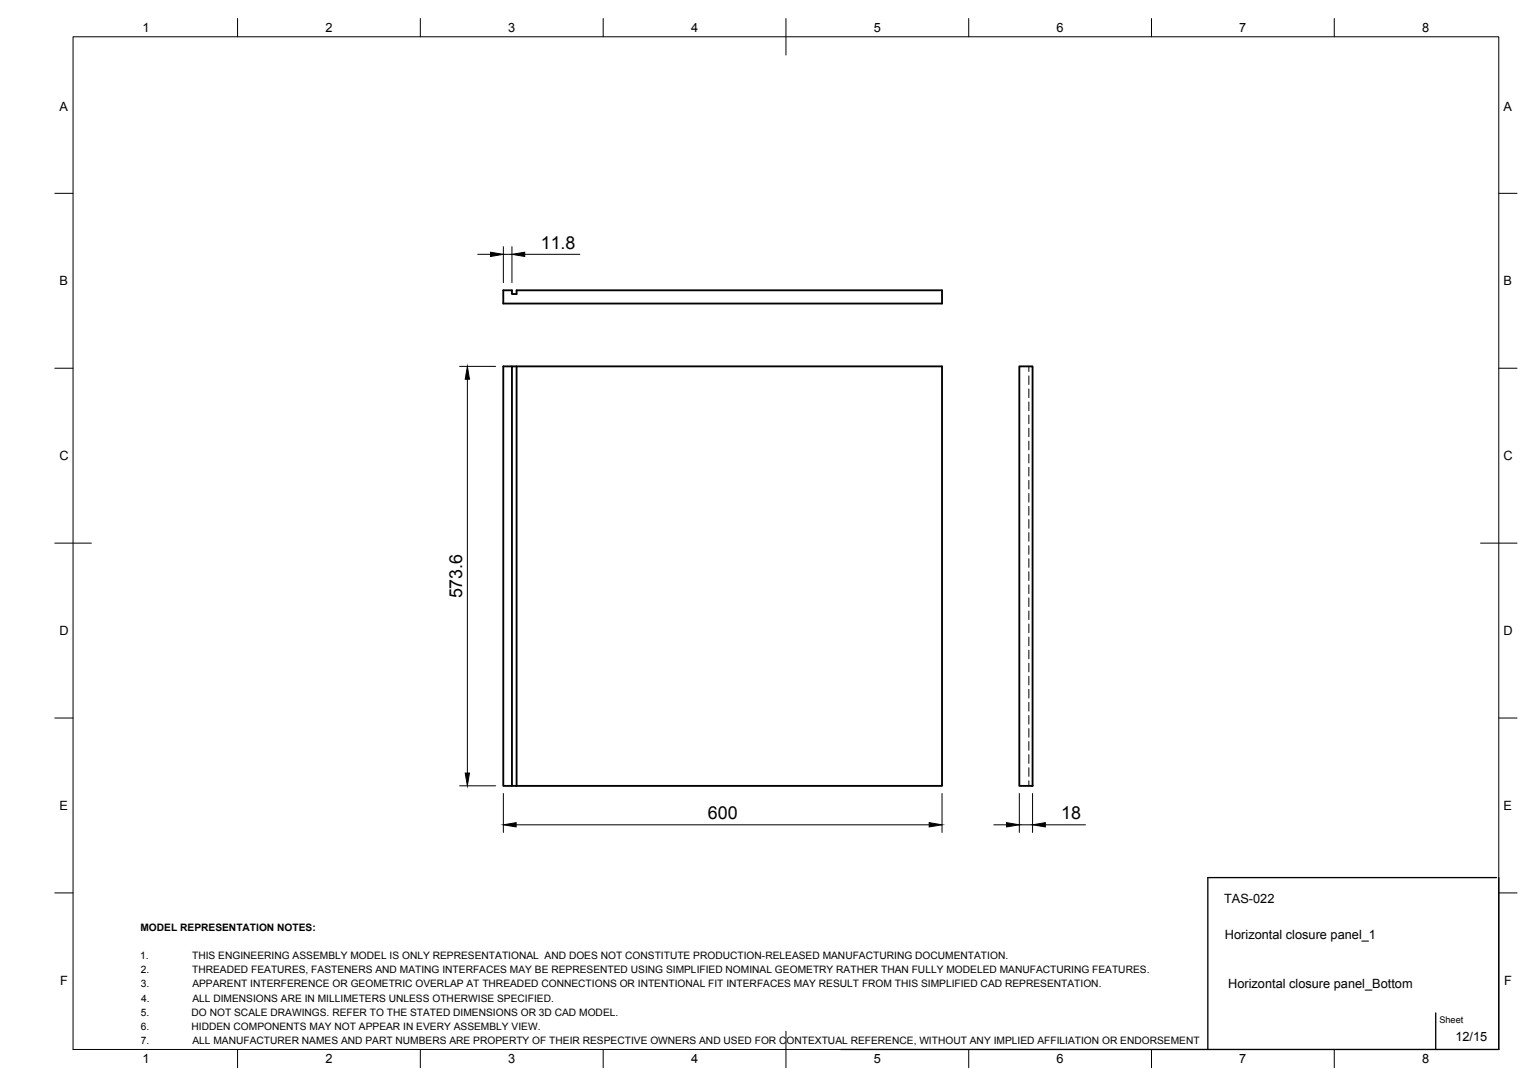
ISO-10303-21;
HEADER;
/* Generated by software containing ST-Developer
 * from STEP Tools, Inc. (www.steptools.com) 
 */

FILE_DESCRIPTION(
/* description */ (''),
/* implementation_level */ '2;1');

FILE_NAME(
/* name */ 'Horizontal closure panel_Bottom.step',
/* time_stamp */ '2026-11-15T21:02:08-08:00',
/* author */ (''),
/* organization */ (''),
/* preprocessor_version */ 'ST-DEVELOPER v20.2',
/* originating_system */ 'Autodesk Translation Framework v15.17.0.0',
/* authorisation */ '');

FILE_SCHEMA (('AUTOMOTIVE_DESIGN { 1 0 10303 214 3 1 1 }'));
ENDSEC;

DATA;
#10=MECHANICAL_DESIGN_GEOMETRIC_PRESENTATION_REPRESENTATION('',(#614),#31566);
#584=SHAPE_REPRESENTATION_RELATIONSHIP('SRR','None',#31648,#599);
#599=ADVANCED_BREP_SHAPE_REPRESENTATION('',(#629),#31563);
#614=STYLED_ITEM('',(#31724),#629);
#629=MANIFOLD_SOLID_BREP('Body1',#5727);
#882=FACE_OUTER_BOUND('',#1187,.T.);
#883=FACE_OUTER_BOUND('',#1188,.T.);
#884=FACE_OUTER_BOUND('',#1189,.T.);
#885=FACE_OUTER_BOUND('',#1190,.T.);
#886=FACE_OUTER_BOUND('',#1191,.T.);
#887=FACE_OUTER_BOUND('',#1192,.T.);
#888=FACE_OUTER_BOUND('',#1193,.T.);
#889=FACE_OUTER_BOUND('',#1194,.T.);
#890=FACE_OUTER_BOUND('',#1195,.T.);
#891=FACE_OUTER_BOUND('',#1196,.T.);
#1187=EDGE_LOOP('',(#5185,#5186,#5187,#5188));
#1188=EDGE_LOOP('',(#5189,#5190,#5191,#5192));
#1189=EDGE_LOOP('',(#5193,#5194,#5195,#5196));
#1190=EDGE_LOOP('',(#5197,#5198,#5199,#5200,#5201,#5202,#5203,#5204));
#1191=EDGE_LOOP('',(#5205,#5206,#5207,#5208));
#1192=EDGE_LOOP('',(#5209,#5210,#5211,#5212));
#1193=EDGE_LOOP('',(#5213,#5214,#5215,#5216));
#1194=EDGE_LOOP('',(#5217,#5218,#5219,#5220,#5221,#5222,#5223,#5224));
#1195=EDGE_LOOP('',(#5225,#5226,#5227,#5228));
#1196=EDGE_LOOP('',(#5229,#5230,#5231,#5232));
#1676=LINE('',#31418,#2183);
#1677=LINE('',#31420,#2184);
#1678=LINE('',#31422,#2185);
#1679=LINE('',#31423,#2186);
#1680=LINE('',#31427,#2187);
#1681=LINE('',#31429,#2188);
#1682=LINE('',#31431,#2189);
#1683=LINE('',#31432,#2190);
#1684=LINE('',#31434,#2191);
#1685=LINE('',#31435,#2192);
#1686=LINE('',#31438,#2193);
#1687=LINE('',#31440,#2194);
#1688=LINE('',#31442,#2195);
#1689=LINE('',#31444,#2196);
#1690=LINE('',#31445,#2197);
#1691=LINE('',#31448,#2198);
#1692=LINE('',#31449,#2199);
#1693=LINE('',#31452,#2200);
#1694=LINE('',#31454,#2201);
#1695=LINE('',#31455,#2202);
#1696=LINE('',#31458,#2203);
#1697=LINE('',#31459,#2204);
#1698=LINE('',#31461,#2205);
#1699=LINE('',#31462,#2206);
#2183=VECTOR('',#7416,1.);
#2184=VECTOR('',#7417,1.);
#2185=VECTOR('',#7418,1.);
#2186=VECTOR('',#7419,1.);
#2187=VECTOR('',#7422,1.);
#2188=VECTOR('',#7423,1.);
#2189=VECTOR('',#7424,1.);
#2190=VECTOR('',#7425,1.);
#2191=VECTOR('',#7428,1.);
#2192=VECTOR('',#7429,1.);
#2193=VECTOR('',#7432,1.);
#2194=VECTOR('',#7433,1.);
#2195=VECTOR('',#7434,1.);
#2196=VECTOR('',#7435,1.);
#2197=VECTOR('',#7436,1.);
#2198=VECTOR('',#7439,1.);
#2199=VECTOR('',#7440,1.);
#2200=VECTOR('',#7443,1.);
#2201=VECTOR('',#7444,1.);
#2202=VECTOR('',#7445,1.);
#2203=VECTOR('',#7448,1.);
#2204=VECTOR('',#7449,1.);
#2205=VECTOR('',#7452,1.);
#2206=VECTOR('',#7453,1.);
#2783=VERTEX_POINT('',#31416);
#2784=VERTEX_POINT('',#31417);
#2785=VERTEX_POINT('',#31419);
#2786=VERTEX_POINT('',#31421);
#2787=VERTEX_POINT('',#31425);
#2788=VERTEX_POINT('',#31426);
#2789=VERTEX_POINT('',#31428);
#2790=VERTEX_POINT('',#31430);
#2791=VERTEX_POINT('',#31437);
#2792=VERTEX_POINT('',#31439);
#2793=VERTEX_POINT('',#31441);
#2794=VERTEX_POINT('',#31443);
#2795=VERTEX_POINT('',#31447);
#2796=VERTEX_POINT('',#31451);
#2797=VERTEX_POINT('',#31453);
#2798=VERTEX_POINT('',#31457);
#3588=EDGE_CURVE('',#2783,#2784,#1676,.T.);
#3589=EDGE_CURVE('',#2785,#2783,#1677,.T.);
#3590=EDGE_CURVE('',#2786,#2785,#1678,.T.);
#3591=EDGE_CURVE('',#2784,#2786,#1679,.T.);
#3592=EDGE_CURVE('',#2787,#2788,#1680,.T.);
#3593=EDGE_CURVE('',#2789,#2787,#1681,.T.);
#3594=EDGE_CURVE('',#2790,#2789,#1682,.T.);
#3595=EDGE_CURVE('',#2788,#2790,#1683,.T.);
#3596=EDGE_CURVE('',#2786,#2789,#1684,.T.);
#3597=EDGE_CURVE('',#2790,#2785,#1685,.T.);
#3598=EDGE_CURVE('',#2791,#2783,#1686,.T.);
#3599=EDGE_CURVE('',#2792,#2791,#1687,.T.);
#3600=EDGE_CURVE('',#2792,#2793,#1688,.T.);
#3601=EDGE_CURVE('',#2793,#2794,#1689,.T.);
#3602=EDGE_CURVE('',#2788,#2794,#1690,.T.);
#3603=EDGE_CURVE('',#2784,#2795,#1691,.T.);
#3604=EDGE_CURVE('',#2795,#2791,#1692,.T.);
#3605=EDGE_CURVE('',#2793,#2796,#1693,.T.);
#3606=EDGE_CURVE('',#2796,#2797,#1694,.T.);
#3607=EDGE_CURVE('',#2794,#2797,#1695,.T.);
#3608=EDGE_CURVE('',#2798,#2792,#1696,.T.);
#3609=EDGE_CURVE('',#2798,#2795,#1697,.T.);
#3610=EDGE_CURVE('',#2797,#2787,#1698,.T.);
#3611=EDGE_CURVE('',#2796,#2798,#1699,.T.);
#5185=ORIENTED_EDGE('',*,*,#3588,.F.);
#5186=ORIENTED_EDGE('',*,*,#3589,.F.);
#5187=ORIENTED_EDGE('',*,*,#3590,.F.);
#5188=ORIENTED_EDGE('',*,*,#3591,.F.);
#5189=ORIENTED_EDGE('',*,*,#3592,.F.);
#5190=ORIENTED_EDGE('',*,*,#3593,.F.);
#5191=ORIENTED_EDGE('',*,*,#3594,.F.);
#5192=ORIENTED_EDGE('',*,*,#3595,.F.);
#5193=ORIENTED_EDGE('',*,*,#3596,.F.);
#5194=ORIENTED_EDGE('',*,*,#3590,.T.);
#5195=ORIENTED_EDGE('',*,*,#3597,.F.);
#5196=ORIENTED_EDGE('',*,*,#3594,.T.);
#5197=ORIENTED_EDGE('',*,*,#3595,.T.);
#5198=ORIENTED_EDGE('',*,*,#3597,.T.);
#5199=ORIENTED_EDGE('',*,*,#3589,.T.);
#5200=ORIENTED_EDGE('',*,*,#3598,.F.);
#5201=ORIENTED_EDGE('',*,*,#3599,.F.);
#5202=ORIENTED_EDGE('',*,*,#3600,.T.);
#5203=ORIENTED_EDGE('',*,*,#3601,.T.);
#5204=ORIENTED_EDGE('',*,*,#3602,.F.);
#5205=ORIENTED_EDGE('',*,*,#3588,.T.);
#5206=ORIENTED_EDGE('',*,*,#3603,.T.);
#5207=ORIENTED_EDGE('',*,*,#3604,.T.);
#5208=ORIENTED_EDGE('',*,*,#3598,.T.);
#5209=ORIENTED_EDGE('',*,*,#3605,.T.);
#5210=ORIENTED_EDGE('',*,*,#3606,.T.);
#5211=ORIENTED_EDGE('',*,*,#3607,.F.);
#5212=ORIENTED_EDGE('',*,*,#3601,.F.);
#5213=ORIENTED_EDGE('',*,*,#3608,.T.);
#5214=ORIENTED_EDGE('',*,*,#3599,.T.);
#5215=ORIENTED_EDGE('',*,*,#3604,.F.);
#5216=ORIENTED_EDGE('',*,*,#3609,.F.);
#5217=ORIENTED_EDGE('',*,*,#3593,.T.);
#5218=ORIENTED_EDGE('',*,*,#3610,.F.);
#5219=ORIENTED_EDGE('',*,*,#3606,.F.);
#5220=ORIENTED_EDGE('',*,*,#3611,.T.);
#5221=ORIENTED_EDGE('',*,*,#3609,.T.);
#5222=ORIENTED_EDGE('',*,*,#3603,.F.);
#5223=ORIENTED_EDGE('',*,*,#3591,.T.);
#5224=ORIENTED_EDGE('',*,*,#3596,.T.);
#5225=ORIENTED_EDGE('',*,*,#3592,.T.);
#5226=ORIENTED_EDGE('',*,*,#3602,.T.);
#5227=ORIENTED_EDGE('',*,*,#3607,.T.);
#5228=ORIENTED_EDGE('',*,*,#3610,.T.);
#5229=ORIENTED_EDGE('',*,*,#3611,.F.);
#5230=ORIENTED_EDGE('',*,*,#3605,.F.);
#5231=ORIENTED_EDGE('',*,*,#3600,.F.);
#5232=ORIENTED_EDGE('',*,*,#3608,.F.);
#5428=PLANE('',#6227);
#5429=PLANE('',#6228);
#5430=PLANE('',#6229);
#5431=PLANE('',#6230);
#5432=PLANE('',#6231);
#5433=PLANE('',#6232);
#5434=PLANE('',#6233);
#5435=PLANE('',#6234);
#5436=PLANE('',#6235);
#5437=PLANE('',#6236);
#5696=ADVANCED_FACE('',(#882),#5428,.F.);
#5697=ADVANCED_FACE('',(#883),#5429,.F.);
#5698=ADVANCED_FACE('',(#884),#5430,.T.);
#5699=ADVANCED_FACE('',(#885),#5431,.T.);
#5700=ADVANCED_FACE('',(#886),#5432,.T.);
#5701=ADVANCED_FACE('',(#887),#5433,.T.);
#5702=ADVANCED_FACE('',(#888),#5434,.T.);
#5703=ADVANCED_FACE('',(#889),#5435,.T.);
#5704=ADVANCED_FACE('',(#890),#5436,.T.);
#5705=ADVANCED_FACE('',(#891),#5437,.F.);
#5727=CLOSED_SHELL('',(#5696,#5697,#5698,#5699,#5700,#5701,#5702,#5703,
#5704,#5705));
#6226=AXIS2_PLACEMENT_3D('',#31414,#7412,#7413);
#6227=AXIS2_PLACEMENT_3D('',#31415,#7414,#7415);
#6228=AXIS2_PLACEMENT_3D('',#31424,#7420,#7421);
#6229=AXIS2_PLACEMENT_3D('',#31433,#7426,#7427);
#6230=AXIS2_PLACEMENT_3D('',#31436,#7430,#7431);
#6231=AXIS2_PLACEMENT_3D('',#31446,#7437,#7438);
#6232=AXIS2_PLACEMENT_3D('',#31450,#7441,#7442);
#6233=AXIS2_PLACEMENT_3D('',#31456,#7446,#7447);
#6234=AXIS2_PLACEMENT_3D('',#31460,#7450,#7451);
#6235=AXIS2_PLACEMENT_3D('',#31463,#7454,#7455);
#6236=AXIS2_PLACEMENT_3D('',#31464,#7456,#7457);
#7412=DIRECTION('axis',(0.,0.,1.));
#7413=DIRECTION('refdir',(1.,0.,0.));
#7414=DIRECTION('center_axis',(0.,-1.,0.));
#7415=DIRECTION('ref_axis',(1.,0.,0.));
#7416=DIRECTION('',(-1.,0.,0.));
#7417=DIRECTION('',(0.,0.,1.));
#7418=DIRECTION('',(1.,0.,0.));
#7419=DIRECTION('',(0.,0.,-1.));
#7420=DIRECTION('center_axis',(0.,1.,0.));
#7421=DIRECTION('ref_axis',(-1.,0.,0.));
#7422=DIRECTION('',(1.,0.,0.));
#7423=DIRECTION('',(0.,0.,1.));
#7424=DIRECTION('',(-1.,0.,0.));
#7425=DIRECTION('',(0.,0.,-1.));
#7426=DIRECTION('center_axis',(0.,0.,1.));
#7427=DIRECTION('ref_axis',(1.,0.,0.));
#7428=DIRECTION('',(0.,1.,0.));
#7429=DIRECTION('',(0.,-1.,0.));
#7430=DIRECTION('center_axis',(1.,0.,0.));
#7431=DIRECTION('ref_axis',(0.,1.,0.));
#7432=DIRECTION('',(0.,1.,0.));
#7433=DIRECTION('',(0.,0.,1.));
#7434=DIRECTION('',(0.,1.,0.));
#7435=DIRECTION('',(0.,0.,1.));
#7436=DIRECTION('',(0.,1.,0.));
#7437=DIRECTION('center_axis',(0.,0.,1.));
#7438=DIRECTION('ref_axis',(1.,0.,0.));
#7439=DIRECTION('',(0.,-1.,0.));
#7440=DIRECTION('',(1.,0.,0.));
#7441=DIRECTION('center_axis',(0.,1.,0.));
#7442=DIRECTION('ref_axis',(-1.,0.,0.));
#7443=DIRECTION('',(-1.,0.,0.));
#7444=DIRECTION('',(0.,0.,1.));
#7445=DIRECTION('',(-1.,0.,0.));
#7446=DIRECTION('center_axis',(0.,-1.,0.));
#7447=DIRECTION('ref_axis',(1.,0.,0.));
#7448=DIRECTION('',(1.,0.,0.));
#7449=DIRECTION('',(0.,0.,1.));
#7450=DIRECTION('center_axis',(-1.,0.,0.));
#7451=DIRECTION('ref_axis',(0.,-1.,0.));
#7452=DIRECTION('',(0.,-1.,0.));
#7453=DIRECTION('',(0.,-1.,0.));
#7454=DIRECTION('center_axis',(0.,0.,1.));
#7455=DIRECTION('ref_axis',(1.,0.,0.));
#7456=DIRECTION('center_axis',(0.,0.,1.));
#7457=DIRECTION('ref_axis',(1.,0.,0.));
#31414=CARTESIAN_POINT('',(0.,0.,0.));
#31415=CARTESIAN_POINT('Origin',(0.,58.18,1.3));
#31416=CARTESIAN_POINT('',(57.36,58.18,1.8));
#31417=CARTESIAN_POINT('',(0.,58.18,1.8));
#31418=CARTESIAN_POINT('',(14.34,58.18,1.8));
#31419=CARTESIAN_POINT('',(57.36,58.18,1.3));
#31420=CARTESIAN_POINT('',(57.36,58.18,0.65));
#31421=CARTESIAN_POINT('',(0.,58.18,1.3));
#31422=CARTESIAN_POINT('',(0.,58.18,1.3));
#31423=CARTESIAN_POINT('',(0.,58.18,0.65));
#31424=CARTESIAN_POINT('Origin',(57.36,58.82,1.3));
#31425=CARTESIAN_POINT('',(0.,58.82,1.8));
#31426=CARTESIAN_POINT('',(57.36,58.82,1.8));
#31427=CARTESIAN_POINT('',(43.02,58.82,1.8));
#31428=CARTESIAN_POINT('',(0.,58.82,1.3));
#31429=CARTESIAN_POINT('',(0.,58.82,0.65));
#31430=CARTESIAN_POINT('',(57.36,58.82,1.3));
#31431=CARTESIAN_POINT('',(57.36,58.82,1.3));
#31432=CARTESIAN_POINT('',(57.36,58.82,0.65));
#31433=CARTESIAN_POINT('Origin',(28.68,58.5,1.3));
#31434=CARTESIAN_POINT('',(0.,59.25,1.3));
#31435=CARTESIAN_POINT('',(57.36,29.25,1.3));
#31436=CARTESIAN_POINT('Origin',(57.36,0.,0.));
#31437=CARTESIAN_POINT('',(57.36,0.,1.8));
#31438=CARTESIAN_POINT('',(57.36,0.,1.8));
#31439=CARTESIAN_POINT('',(57.36,0.,0.));
#31440=CARTESIAN_POINT('',(57.36,0.,0.));
#31441=CARTESIAN_POINT('',(57.36,60.,0.));
#31442=CARTESIAN_POINT('',(57.36,0.,0.));
#31443=CARTESIAN_POINT('',(57.36,60.,1.8));
#31444=CARTESIAN_POINT('',(57.36,60.,0.));
#31445=CARTESIAN_POINT('',(57.36,0.,1.8));
#31446=CARTESIAN_POINT('Origin',(28.68,30.,1.8));
#31447=CARTESIAN_POINT('',(0.,0.,1.8));
#31448=CARTESIAN_POINT('',(0.,60.,1.8));
#31449=CARTESIAN_POINT('',(0.,0.,1.8));
#31450=CARTESIAN_POINT('Origin',(57.36,60.,0.));
#31451=CARTESIAN_POINT('',(0.,60.,0.));
#31452=CARTESIAN_POINT('',(57.36,60.,0.));
#31453=CARTESIAN_POINT('',(0.,60.,1.8));
#31454=CARTESIAN_POINT('',(0.,60.,0.));
#31455=CARTESIAN_POINT('',(57.36,60.,1.8));
#31456=CARTESIAN_POINT('Origin',(0.,0.,0.));
#31457=CARTESIAN_POINT('',(0.,0.,0.));
#31458=CARTESIAN_POINT('',(0.,0.,0.));
#31459=CARTESIAN_POINT('',(0.,0.,0.));
#31460=CARTESIAN_POINT('Origin',(0.,60.,0.));
#31461=CARTESIAN_POINT('',(0.,60.,1.8));
#31462=CARTESIAN_POINT('',(0.,60.,0.));
#31463=CARTESIAN_POINT('Origin',(28.68,30.,1.8));
#31464=CARTESIAN_POINT('Origin',(28.68,30.,0.));
#31546=UNCERTAINTY_MEASURE_WITH_UNIT(LENGTH_MEASURE(0.001),#31567,
'DISTANCE_ACCURACY_VALUE',
'Maximum model space distance between geometric entities at asserted c
onnectivities');
#31549=UNCERTAINTY_MEASURE_WITH_UNIT(LENGTH_MEASURE(0.001),#31567,
'DISTANCE_ACCURACY_VALUE',
'Maximum model space distance between geometric entities at asserted c
onnectivities');
#31563=(
GEOMETRIC_REPRESENTATION_CONTEXT(3)
GLOBAL_UNCERTAINTY_ASSIGNED_CONTEXT((#31546))
GLOBAL_UNIT_ASSIGNED_CONTEXT((#31567,#31569,#31570))
REPRESENTATION_CONTEXT('','3D')
);
#31566=(
GEOMETRIC_REPRESENTATION_CONTEXT(3)
GLOBAL_UNCERTAINTY_ASSIGNED_CONTEXT((#31549))
GLOBAL_UNIT_ASSIGNED_CONTEXT((#31567,#31569,#31570))
REPRESENTATION_CONTEXT('','3D')
);
#31567=(
LENGTH_UNIT()
NAMED_UNIT(*)
SI_UNIT(.CENTI.,.METRE.)
);
#31569=(
NAMED_UNIT(*)
PLANE_ANGLE_UNIT()
SI_UNIT($,.RADIAN.)
);
#31570=(
NAMED_UNIT(*)
SI_UNIT($,.STERADIAN.)
SOLID_ANGLE_UNIT()
);
#31584=SHAPE_DEFINITION_REPRESENTATION(#31600,#31648);
#31600=PRODUCT_DEFINITION_SHAPE('',$,#31665);
#31648=SHAPE_REPRESENTATION('',(#6226),#31563);
#31651=PRODUCT_DEFINITION_CONTEXT('part definition',#31701,'design');
#31665=PRODUCT_DEFINITION('Horizontal closure panel_1',
'Horizontal closure panel_Bottom',#31681,#31651);
#31681=PRODUCT_DEFINITION_FORMATION('',$,#31716);
#31701=APPLICATION_CONTEXT(
'Core Data for Automotive Mechanical Design Process');
#31702=PRODUCT_CONTEXT('part definition',#31701,'mechanical');
#31716=PRODUCT('Horizontal closure panel_1',
'Horizontal closure panel_Bottom',$,(#31702));
#31724=PRESENTATION_STYLE_ASSIGNMENT((#31731));
#31731=SURFACE_STYLE_USAGE(.BOTH.,#31738);
#31738=SURFACE_SIDE_STYLE('',(#31745));
#31745=SURFACE_STYLE_FILL_AREA(#31752);
#31752=FILL_AREA_STYLE('Opaque(169,210,234)',(#31759));
#31759=FILL_AREA_STYLE_COLOUR('Opaque(169,210,234)',#31766);
#31766=COLOUR_RGB('Opaque(169,210,234)',0.662745098039216,0.823529411764706,
0.917647058823529);
ENDSEC;
END-ISO-10303-21;
